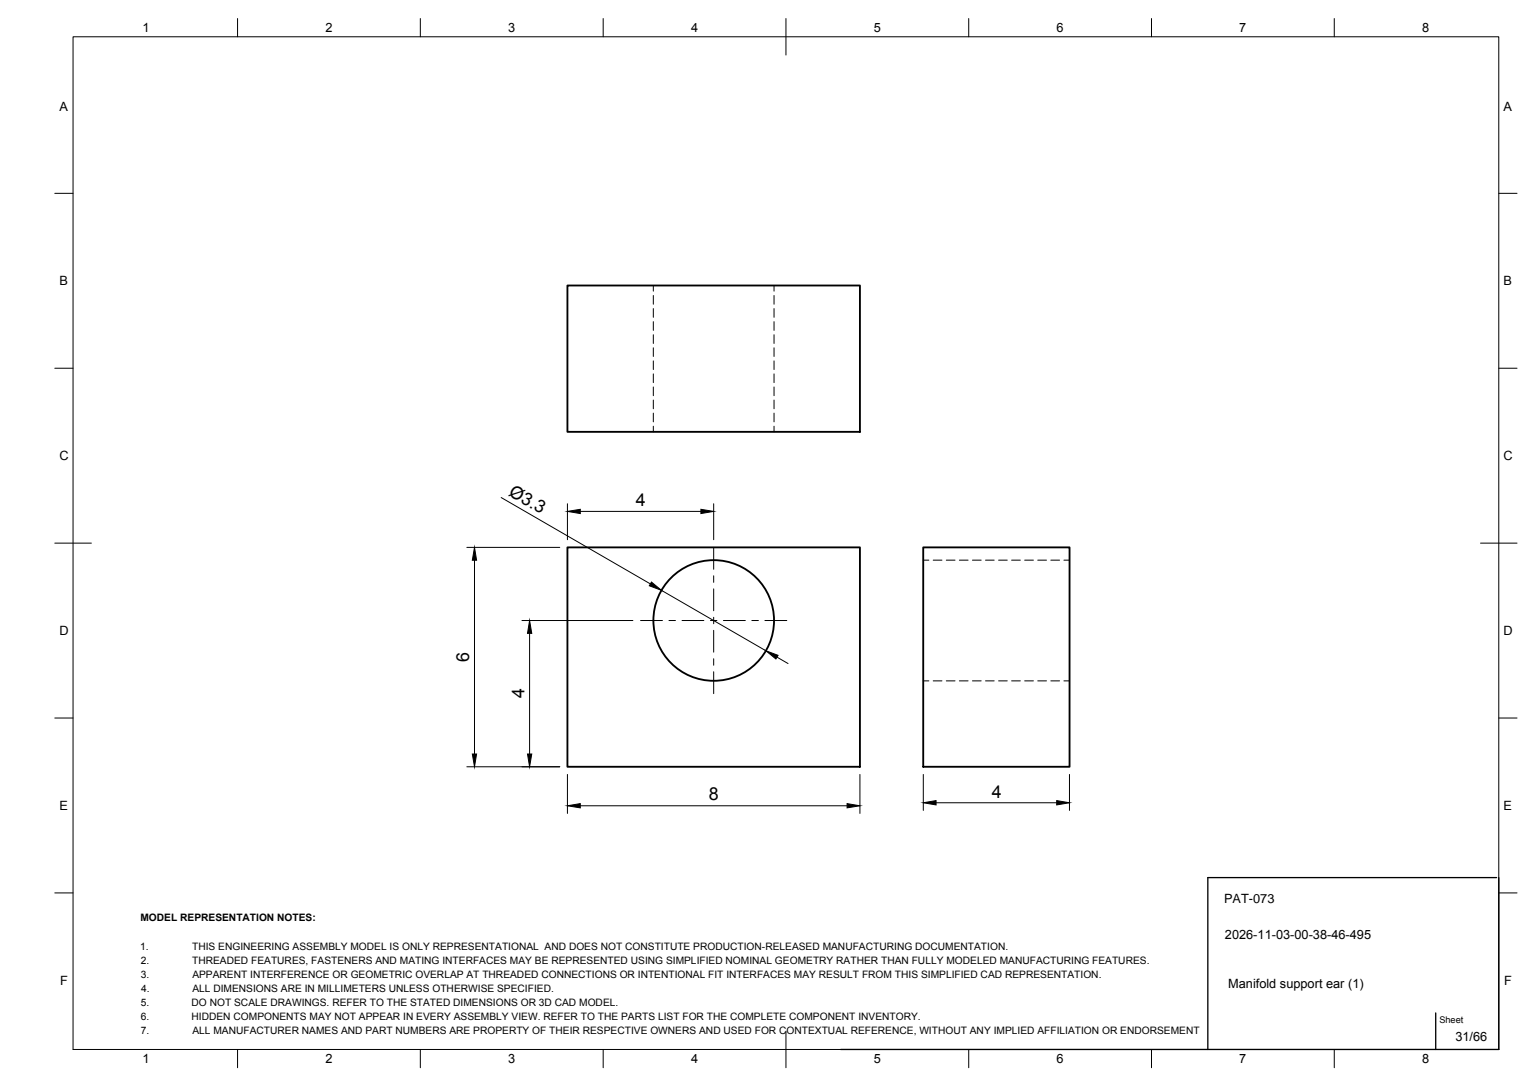
ISO-10303-21;
HEADER;
/* Generated by software containing ST-Developer
 * from STEP Tools, Inc. (www.steptools.com) 
 */

FILE_DESCRIPTION(
/* description */ ('Manual piston pump'),
/* implementation_level */ '2;1');

FILE_NAME(
/* name */ 'Manifold support ear (1).step',
/* time_stamp */ '2026-11-02T16:54:23-08:00',
/* author */ (''),
/* organization */ (''),
/* preprocessor_version */ 'ST-DEVELOPER v20.2',
/* originating_system */ 'Autodesk Translation Framework v15.17.0.0',
/* authorisation */ '');

FILE_SCHEMA (('AUTOMOTIVE_DESIGN { 1 0 10303 214 3 1 1 }'));
ENDSEC;

DATA;
#10=MECHANICAL_DESIGN_GEOMETRIC_PRESENTATION_REPRESENTATION('',(#733),#19043);
#599=SHAPE_REPRESENTATION_RELATIONSHIP('SRR','None',#19347,#662);
#662=ADVANCED_BREP_SHAPE_REPRESENTATION('',(#803),#19014);
#733=STYLED_ITEM('',(#19661),#803);
#803=MANIFOLD_SOLID_BREP('Body1',#9519);
#995=FACE_BOUND('',#2420,.T.);
#996=FACE_BOUND('',#2422,.T.);
#1231=CYLINDRICAL_SURFACE('',#11022,0.165);
#1671=FACE_OUTER_BOUND('',#2414,.T.);
#1672=FACE_OUTER_BOUND('',#2415,.T.);
#1673=FACE_OUTER_BOUND('',#2416,.T.);
#1674=FACE_OUTER_BOUND('',#2417,.T.);
#1675=FACE_OUTER_BOUND('',#2418,.T.);
#1676=FACE_OUTER_BOUND('',#2419,.T.);
#1677=FACE_OUTER_BOUND('',#2421,.T.);
#2414=EDGE_LOOP('',(#7829,#7830,#7831,#7832));
#2415=EDGE_LOOP('',(#7833,#7834,#7835,#7836));
#2416=EDGE_LOOP('',(#7837,#7838,#7839,#7840));
#2417=EDGE_LOOP('',(#7841,#7842,#7843,#7844));
#2418=EDGE_LOOP('',(#7845,#7846,#7847,#7848));
#2419=EDGE_LOOP('',(#7849,#7850,#7851,#7852));
#2420=EDGE_LOOP('',(#7853));
#2421=EDGE_LOOP('',(#7854,#7855,#7856,#7857));
#2422=EDGE_LOOP('',(#7858));
#3009=CIRCLE('',#11023,0.165);
#3010=CIRCLE('',#11024,0.165);
#3533=LINE('',#17828,#4137);
#3534=LINE('',#17833,#4138);
#3535=LINE('',#17835,#4139);
#3536=LINE('',#17837,#4140);
#3537=LINE('',#17838,#4141);
#3538=LINE('',#17841,#4142);
#3539=LINE('',#17843,#4143);
#3540=LINE('',#17844,#4144);
#3541=LINE('',#17847,#4145);
#3542=LINE('',#17849,#4146);
#3543=LINE('',#17850,#4147);
#3544=LINE('',#17852,#4148);
#3545=LINE('',#17853,#4149);
#4137=VECTOR('',#13443,0.165);
#4138=VECTOR('',#13448,1.);
#4139=VECTOR('',#13449,1.);
#4140=VECTOR('',#13450,1.);
#4141=VECTOR('',#13451,1.);
#4142=VECTOR('',#13454,1.);
#4143=VECTOR('',#13455,1.);
#4144=VECTOR('',#13456,1.);
#4145=VECTOR('',#13459,1.);
#4146=VECTOR('',#13460,1.);
#4147=VECTOR('',#13461,1.);
#4148=VECTOR('',#13464,1.);
#4149=VECTOR('',#13465,1.);
#4880=VERTEX_POINT('',#17825);
#4881=VERTEX_POINT('',#17827);
#4882=VERTEX_POINT('',#17831);
#4883=VERTEX_POINT('',#17832);
#4884=VERTEX_POINT('',#17834);
#4885=VERTEX_POINT('',#17836);
#4886=VERTEX_POINT('',#17840);
#4887=VERTEX_POINT('',#17842);
#4888=VERTEX_POINT('',#17846);
#4889=VERTEX_POINT('',#17848);
#5901=EDGE_CURVE('',#4880,#4880,#3009,.T.);
#5902=EDGE_CURVE('',#4880,#4881,#3533,.T.);
#5903=EDGE_CURVE('',#4881,#4881,#3010,.T.);
#5904=EDGE_CURVE('',#4882,#4883,#3534,.T.);
#5905=EDGE_CURVE('',#4883,#4884,#3535,.T.);
#5906=EDGE_CURVE('',#4885,#4884,#3536,.T.);
#5907=EDGE_CURVE('',#4882,#4885,#3537,.T.);
#5908=EDGE_CURVE('',#4886,#4882,#3538,.T.);
#5909=EDGE_CURVE('',#4887,#4885,#3539,.T.);
#5910=EDGE_CURVE('',#4886,#4887,#3540,.T.);
#5911=EDGE_CURVE('',#4888,#4886,#3541,.T.);
#5912=EDGE_CURVE('',#4889,#4887,#3542,.T.);
#5913=EDGE_CURVE('',#4888,#4889,#3543,.T.);
#5914=EDGE_CURVE('',#4883,#4888,#3544,.T.);
#5915=EDGE_CURVE('',#4884,#4889,#3545,.T.);
#7829=ORIENTED_EDGE('',*,*,#5901,.F.);
#7830=ORIENTED_EDGE('',*,*,#5902,.T.);
#7831=ORIENTED_EDGE('',*,*,#5903,.F.);
#7832=ORIENTED_EDGE('',*,*,#5902,.F.);
#7833=ORIENTED_EDGE('',*,*,#5904,.T.);
#7834=ORIENTED_EDGE('',*,*,#5905,.T.);
#7835=ORIENTED_EDGE('',*,*,#5906,.F.);
#7836=ORIENTED_EDGE('',*,*,#5907,.F.);
#7837=ORIENTED_EDGE('',*,*,#5908,.T.);
#7838=ORIENTED_EDGE('',*,*,#5907,.T.);
#7839=ORIENTED_EDGE('',*,*,#5909,.F.);
#7840=ORIENTED_EDGE('',*,*,#5910,.F.);
#7841=ORIENTED_EDGE('',*,*,#5911,.T.);
#7842=ORIENTED_EDGE('',*,*,#5910,.T.);
#7843=ORIENTED_EDGE('',*,*,#5912,.F.);
#7844=ORIENTED_EDGE('',*,*,#5913,.F.);
#7845=ORIENTED_EDGE('',*,*,#5914,.T.);
#7846=ORIENTED_EDGE('',*,*,#5913,.T.);
#7847=ORIENTED_EDGE('',*,*,#5915,.F.);
#7848=ORIENTED_EDGE('',*,*,#5905,.F.);
#7849=ORIENTED_EDGE('',*,*,#5915,.T.);
#7850=ORIENTED_EDGE('',*,*,#5912,.T.);
#7851=ORIENTED_EDGE('',*,*,#5909,.T.);
#7852=ORIENTED_EDGE('',*,*,#5906,.T.);
#7853=ORIENTED_EDGE('',*,*,#5903,.T.);
#7854=ORIENTED_EDGE('',*,*,#5914,.F.);
#7855=ORIENTED_EDGE('',*,*,#5904,.F.);
#7856=ORIENTED_EDGE('',*,*,#5908,.F.);
#7857=ORIENTED_EDGE('',*,*,#5911,.F.);
#7858=ORIENTED_EDGE('',*,*,#5901,.T.);
#8775=PLANE('',#11025);
#8776=PLANE('',#11026);
#8777=PLANE('',#11027);
#8778=PLANE('',#11028);
#8779=PLANE('',#11029);
#8780=PLANE('',#11030);
#9276=ADVANCED_FACE('',(#1671),#1231,.F.);
#9277=ADVANCED_FACE('',(#1672),#8775,.T.);
#9278=ADVANCED_FACE('',(#1673),#8776,.T.);
#9279=ADVANCED_FACE('',(#1674),#8777,.T.);
#9280=ADVANCED_FACE('',(#1675),#8778,.T.);
#9281=ADVANCED_FACE('',(#1676,#995),#8779,.T.);
#9282=ADVANCED_FACE('',(#1677,#996),#8780,.F.);
#9519=CLOSED_SHELL('',(#9276,#9277,#9278,#9279,#9280,#9281,#9282));
#11021=AXIS2_PLACEMENT_3D('',#17823,#13437,#13438);
#11022=AXIS2_PLACEMENT_3D('',#17824,#13439,#13440);
#11023=AXIS2_PLACEMENT_3D('',#17826,#13441,#13442);
#11024=AXIS2_PLACEMENT_3D('',#17829,#13444,#13445);
#11025=AXIS2_PLACEMENT_3D('',#17830,#13446,#13447);
#11026=AXIS2_PLACEMENT_3D('',#17839,#13452,#13453);
#11027=AXIS2_PLACEMENT_3D('',#17845,#13457,#13458);
#11028=AXIS2_PLACEMENT_3D('',#17851,#13462,#13463);
#11029=AXIS2_PLACEMENT_3D('',#17854,#13466,#13467);
#11030=AXIS2_PLACEMENT_3D('',#17855,#13468,#13469);
#13437=DIRECTION('axis',(0.,0.,1.));
#13438=DIRECTION('refdir',(1.,0.,0.));
#13439=DIRECTION('center_axis',(0.,0.,1.));
#13440=DIRECTION('ref_axis',(1.,0.,0.));
#13441=DIRECTION('center_axis',(0.,0.,1.));
#13442=DIRECTION('ref_axis',(1.,0.,0.));
#13443=DIRECTION('',(0.,0.,1.));
#13444=DIRECTION('center_axis',(0.,0.,-1.));
#13445=DIRECTION('ref_axis',(1.,0.,0.));
#13446=DIRECTION('center_axis',(0.,1.,0.));
#13447=DIRECTION('ref_axis',(-1.,0.,0.));
#13448=DIRECTION('',(-1.,0.,0.));
#13449=DIRECTION('',(0.,0.,1.));
#13450=DIRECTION('',(-1.,0.,0.));
#13451=DIRECTION('',(0.,0.,1.));
#13452=DIRECTION('center_axis',(1.,0.,0.));
#13453=DIRECTION('ref_axis',(0.,1.,0.));
#13454=DIRECTION('',(0.,1.,0.));
#13455=DIRECTION('',(0.,1.,0.));
#13456=DIRECTION('',(0.,0.,1.));
#13457=DIRECTION('center_axis',(0.,-1.,0.));
#13458=DIRECTION('ref_axis',(1.,0.,0.));
#13459=DIRECTION('',(1.,0.,0.));
#13460=DIRECTION('',(1.,0.,0.));
#13461=DIRECTION('',(0.,0.,1.));
#13462=DIRECTION('center_axis',(-1.,0.,0.));
#13463=DIRECTION('ref_axis',(0.,-1.,0.));
#13464=DIRECTION('',(0.,-1.,0.));
#13465=DIRECTION('',(0.,-1.,0.));
#13466=DIRECTION('center_axis',(0.,0.,1.));
#13467=DIRECTION('ref_axis',(1.,0.,0.));
#13468=DIRECTION('center_axis',(0.,0.,1.));
#13469=DIRECTION('ref_axis',(1.,0.,0.));
#17823=CARTESIAN_POINT('',(0.,0.,0.));
#17824=CARTESIAN_POINT('Origin',(0.7,10.7,6.5));
#17825=CARTESIAN_POINT('',(0.535,10.7,6.6));
#17826=CARTESIAN_POINT('Origin',(0.7,10.7,6.6));
#17827=CARTESIAN_POINT('',(0.535,10.7,7.));
#17828=CARTESIAN_POINT('',(0.535,10.7,6.5));
#17829=CARTESIAN_POINT('Origin',(0.7,10.7,7.));
#17830=CARTESIAN_POINT('Origin',(1.1,10.9,6.6));
#17831=CARTESIAN_POINT('',(1.1,10.9,6.6));
#17832=CARTESIAN_POINT('',(0.3,10.9,6.6));
#17833=CARTESIAN_POINT('',(1.1,10.9,6.6));
#17834=CARTESIAN_POINT('',(0.3,10.9,7.));
#17835=CARTESIAN_POINT('',(0.3,10.9,6.6));
#17836=CARTESIAN_POINT('',(1.1,10.9,7.));
#17837=CARTESIAN_POINT('',(1.1,10.9,7.));
#17838=CARTESIAN_POINT('',(1.1,10.9,6.6));
#17839=CARTESIAN_POINT('Origin',(1.1,10.3,6.6));
#17840=CARTESIAN_POINT('',(1.1,10.3,6.6));
#17841=CARTESIAN_POINT('',(1.1,10.3,6.6));
#17842=CARTESIAN_POINT('',(1.1,10.3,7.));
#17843=CARTESIAN_POINT('',(1.1,10.3,7.));
#17844=CARTESIAN_POINT('',(1.1,10.3,6.6));
#17845=CARTESIAN_POINT('Origin',(0.3,10.3,6.6));
#17846=CARTESIAN_POINT('',(0.3,10.3,6.6));
#17847=CARTESIAN_POINT('',(0.3,10.3,6.6));
#17848=CARTESIAN_POINT('',(0.3,10.3,7.));
#17849=CARTESIAN_POINT('',(0.3,10.3,7.));
#17850=CARTESIAN_POINT('',(0.3,10.3,6.6));
#17851=CARTESIAN_POINT('Origin',(0.3,10.9,6.6));
#17852=CARTESIAN_POINT('',(0.3,10.9,6.6));
#17853=CARTESIAN_POINT('',(0.3,10.9,7.));
#17854=CARTESIAN_POINT('Origin',(0.7,10.6,7.));
#17855=CARTESIAN_POINT('Origin',(0.7,10.6,6.6));
#18943=UNCERTAINTY_MEASURE_WITH_UNIT(LENGTH_MEASURE(0.001),#19044,
'DISTANCE_ACCURACY_VALUE',
'Maximum model space distance between geometric entities at asserted c
onnectivities');
#18972=UNCERTAINTY_MEASURE_WITH_UNIT(LENGTH_MEASURE(0.001),#19044,
'DISTANCE_ACCURACY_VALUE',
'Maximum model space distance between geometric entities at asserted c
onnectivities');
#19014=(
GEOMETRIC_REPRESENTATION_CONTEXT(3)
GLOBAL_UNCERTAINTY_ASSIGNED_CONTEXT((#18943))
GLOBAL_UNIT_ASSIGNED_CONTEXT((#19044,#19046,#19047))
REPRESENTATION_CONTEXT('','3D')
);
#19043=(
GEOMETRIC_REPRESENTATION_CONTEXT(3)
GLOBAL_UNCERTAINTY_ASSIGNED_CONTEXT((#18972))
GLOBAL_UNIT_ASSIGNED_CONTEXT((#19044,#19046,#19047))
REPRESENTATION_CONTEXT('','3D')
);
#19044=(
LENGTH_UNIT()
NAMED_UNIT(*)
SI_UNIT(.CENTI.,.METRE.)
);
#19046=(
NAMED_UNIT(*)
PLANE_ANGLE_UNIT()
SI_UNIT($,.RADIAN.)
);
#19047=(
NAMED_UNIT(*)
SI_UNIT($,.STERADIAN.)
SOLID_ANGLE_UNIT()
);
#19089=SHAPE_DEFINITION_REPRESENTATION(#19166,#19347);
#19166=PRODUCT_DEFINITION_SHAPE('',$,#19418);
#19347=SHAPE_REPRESENTATION('',(#11021),#19014);
#19376=PRODUCT_DEFINITION_CONTEXT('part definition',#19588,'design');
#19418=PRODUCT_DEFINITION('2026-11-03-00-38-46-495',
'Manifold support ear (1)',#19488,#19376);
#19488=PRODUCT_DEFINITION_FORMATION('',$,#19631);
#19588=APPLICATION_CONTEXT(
'Core Data for Automotive Mechanical Design Process');
#19589=PRODUCT_CONTEXT('part definition',#19588,'mechanical');
#19631=PRODUCT('2026-11-03-00-38-46-495','Manifold support ear (1)',
'Manifold support ear',(#19589));
#19661=PRESENTATION_STYLE_ASSIGNMENT((#19667));
#19667=SURFACE_STYLE_USAGE(.BOTH.,#19673);
#19673=SURFACE_SIDE_STYLE('',(#19679));
#19679=SURFACE_STYLE_FILL_AREA(#19685);
#19685=FILL_AREA_STYLE('CAD Library Painted - Engineering blue',(#19691));
#19691=FILL_AREA_STYLE_COLOUR('CAD Library Painted - Engineering blue',
#19697);
#19697=COLOUR_RGB('CAD Library Painted - Engineering blue',0.12156862745098,
0.356862745098039,0.6);
ENDSEC;
END-ISO-10303-21;
